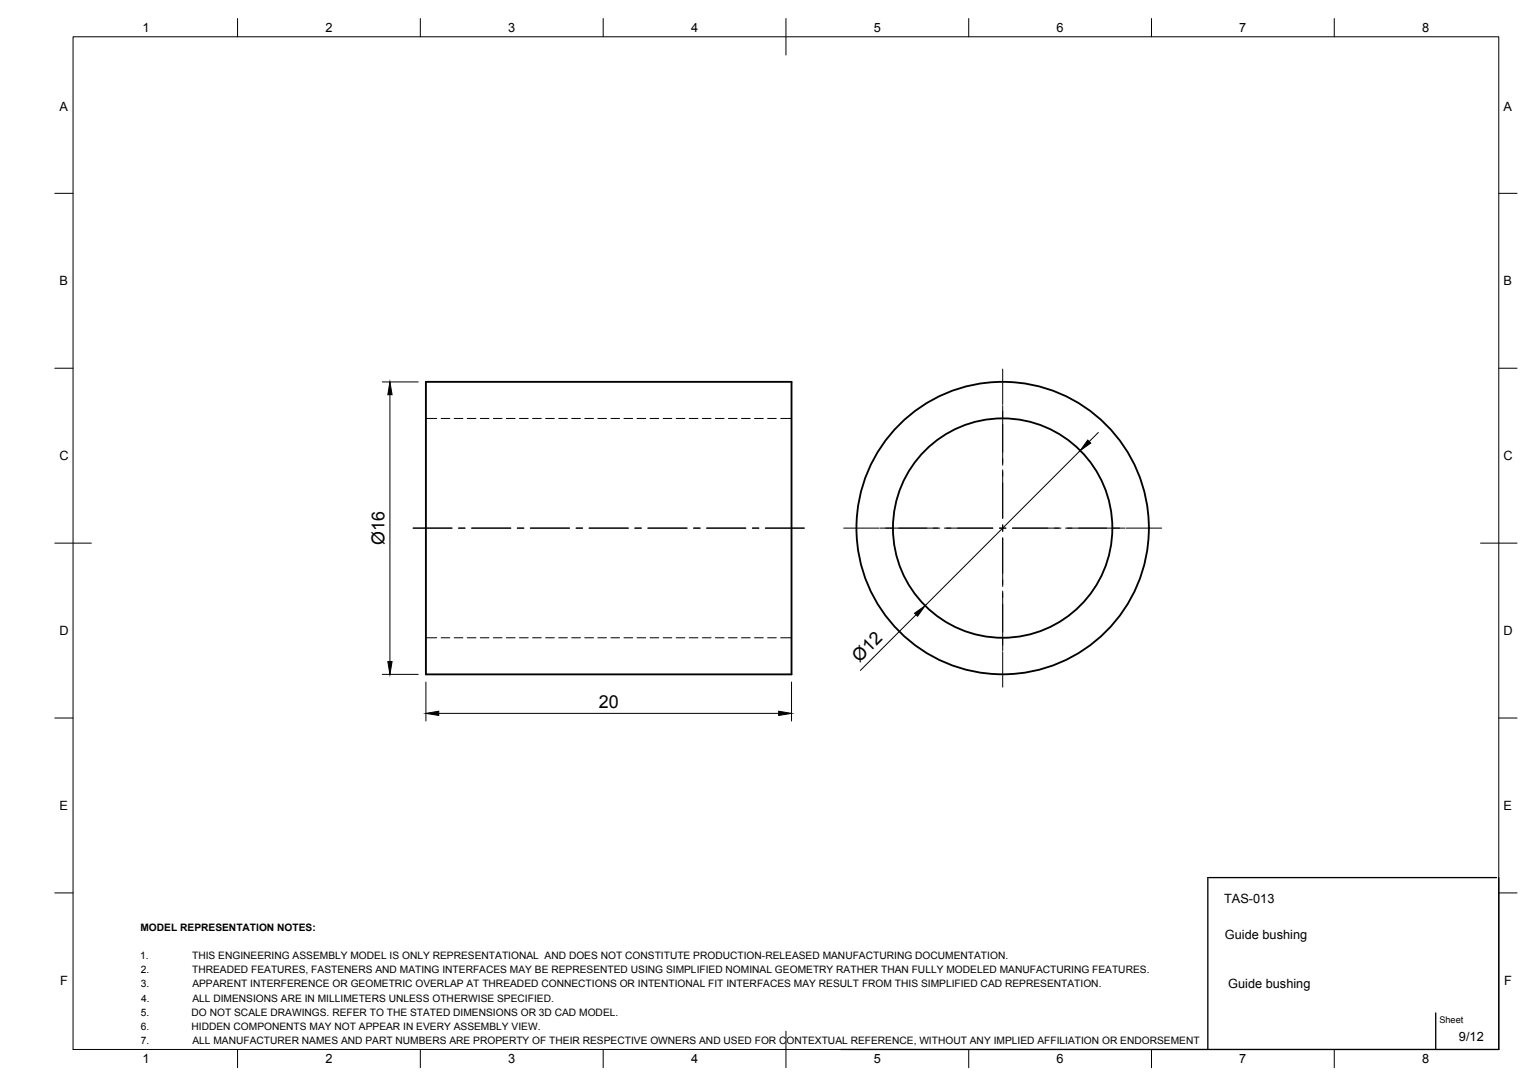
ISO-10303-21;
HEADER;
/* Generated by software containing ST-Developer
 * from STEP Tools, Inc. (www.steptools.com) 
 */

FILE_DESCRIPTION(
/* description */ (
'Independent guided parallel-jaw bracket clamp. Two12mm guide rods, re
placeable bronze sleeves, captured swiveling spindle, replaceable jaw 
pads and modeled M16x2 screw. Native slider/revolute joints linked2mm 
per revolution. Nominal opening0..122 with initial28mm. Base and two i
dentical supports welded. Standard fits, weld details and clamp load r
equire engineering selection.'),
/* implementation_level */ '2;1');

FILE_NAME(
/* name */ 'Guide bushing.step',
/* time_stamp */ '2026-11-14T09:15:44-08:00',
/* author */ (''),
/* organization */ (''),
/* preprocessor_version */ 'ST-DEVELOPER v20.2',
/* originating_system */ 'Autodesk Translation Framework v15.17.0.0',
/* authorisation */ '');

FILE_SCHEMA (('AUTOMOTIVE_DESIGN { 1 0 10303 214 3 1 1 }'));
ENDSEC;

DATA;
#10=MECHANICAL_DESIGN_GEOMETRIC_PRESENTATION_REPRESENTATION('',(#924),#105806);
#900=SHAPE_REPRESENTATION_RELATIONSHIP('SRR','None',#105868,#912);
#912=ADVANCED_BREP_SHAPE_REPRESENTATION('',(#936),#105803);
#924=STYLED_ITEM('',(#105930),#936);
#936=MANIFOLD_SOLID_BREP('Body1',#7211);
#992=FACE_BOUND('',#1617,.T.);
#993=FACE_BOUND('',#1619,.T.);
#1051=PLANE('',#7665);
#1052=PLANE('',#7666);
#1289=FACE_OUTER_BOUND('',#1614,.T.);
#1290=FACE_OUTER_BOUND('',#1615,.T.);
#1291=FACE_OUTER_BOUND('',#1616,.T.);
#1292=FACE_OUTER_BOUND('',#1618,.T.);
#1614=EDGE_LOOP('',(#6341,#6342,#6343,#6344));
#1615=EDGE_LOOP('',(#6345,#6346,#6347,#6348));
#1616=EDGE_LOOP('',(#6349));
#1617=EDGE_LOOP('',(#6350));
#1618=EDGE_LOOP('',(#6351));
#1619=EDGE_LOOP('',(#6352));
#1900=LINE('',#88827,#2180);
#1901=LINE('',#88833,#2181);
#2180=VECTOR('',#8603,6.);
#2181=VECTOR('',#8610,8.);
#2311=CIRCLE('',#7660,6.);
#2312=CIRCLE('',#7661,6.);
#2313=CIRCLE('',#7663,8.);
#2314=CIRCLE('',#7664,8.);
#3093=VERTEX_POINT('',#88824);
#3094=VERTEX_POINT('',#88826);
#3095=VERTEX_POINT('',#88830);
#3096=VERTEX_POINT('',#88832);
#4215=EDGE_CURVE('',#3093,#3093,#2311,.T.);
#4216=EDGE_CURVE('',#3093,#3094,#1900,.T.);
#4217=EDGE_CURVE('',#3094,#3094,#2312,.T.);
#4218=EDGE_CURVE('',#3095,#3095,#2313,.T.);
#4219=EDGE_CURVE('',#3095,#3096,#1901,.T.);
#4220=EDGE_CURVE('',#3096,#3096,#2314,.T.);
#6341=ORIENTED_EDGE('',*,*,#4215,.T.);
#6342=ORIENTED_EDGE('',*,*,#4216,.T.);
#6343=ORIENTED_EDGE('',*,*,#4217,.F.);
#6344=ORIENTED_EDGE('',*,*,#4216,.F.);
#6345=ORIENTED_EDGE('',*,*,#4218,.F.);
#6346=ORIENTED_EDGE('',*,*,#4219,.T.);
#6347=ORIENTED_EDGE('',*,*,#4220,.T.);
#6348=ORIENTED_EDGE('',*,*,#4219,.F.);
#6349=ORIENTED_EDGE('',*,*,#4218,.T.);
#6350=ORIENTED_EDGE('',*,*,#4217,.T.);
#6351=ORIENTED_EDGE('',*,*,#4220,.F.);
#6352=ORIENTED_EDGE('',*,*,#4215,.F.);
#6899=CYLINDRICAL_SURFACE('',#7659,6.);
#6900=CYLINDRICAL_SURFACE('',#7662,8.);
#7154=ADVANCED_FACE('',(#1289),#6899,.F.);
#7155=ADVANCED_FACE('',(#1290),#6900,.T.);
#7156=ADVANCED_FACE('',(#1291,#992),#1051,.T.);
#7157=ADVANCED_FACE('',(#1292,#993),#1052,.F.);
#7211=CLOSED_SHELL('',(#7154,#7155,#7156,#7157));
#7658=AXIS2_PLACEMENT_3D('',#88822,#8597,#8598);
#7659=AXIS2_PLACEMENT_3D('',#88823,#8599,#8600);
#7660=AXIS2_PLACEMENT_3D('',#88825,#8601,#8602);
#7661=AXIS2_PLACEMENT_3D('',#88828,#8604,#8605);
#7662=AXIS2_PLACEMENT_3D('',#88829,#8606,#8607);
#7663=AXIS2_PLACEMENT_3D('',#88831,#8608,#8609);
#7664=AXIS2_PLACEMENT_3D('',#88834,#8611,#8612);
#7665=AXIS2_PLACEMENT_3D('',#88835,#8613,#8614);
#7666=AXIS2_PLACEMENT_3D('',#88836,#8615,#8616);
#8597=DIRECTION('axis',(0.,0.,1.));
#8598=DIRECTION('refdir',(1.,0.,0.));
#8599=DIRECTION('center_axis',(0.,0.,1.));
#8600=DIRECTION('ref_axis',(1.,0.,0.));
#8601=DIRECTION('center_axis',(0.,0.,-1.));
#8602=DIRECTION('ref_axis',(1.,0.,0.));
#8603=DIRECTION('',(0.,0.,1.));
#8604=DIRECTION('center_axis',(0.,0.,-1.));
#8605=DIRECTION('ref_axis',(1.,0.,0.));
#8606=DIRECTION('center_axis',(0.,0.,1.));
#8607=DIRECTION('ref_axis',(1.,0.,0.));
#8608=DIRECTION('center_axis',(0.,0.,1.));
#8609=DIRECTION('ref_axis',(1.,0.,0.));
#8610=DIRECTION('',(0.,0.,-1.));
#8611=DIRECTION('center_axis',(0.,0.,1.));
#8612=DIRECTION('ref_axis',(1.,0.,0.));
#8613=DIRECTION('center_axis',(0.,0.,1.));
#8614=DIRECTION('ref_axis',(1.,0.,0.));
#8615=DIRECTION('center_axis',(0.,0.,1.));
#8616=DIRECTION('ref_axis',(1.,0.,0.));
#88822=CARTESIAN_POINT('',(0.,0.,0.));
#88823=CARTESIAN_POINT('Origin',(0.,0.,0.));
#88824=CARTESIAN_POINT('',(-6.,-7.34788079488412E-16,0.));
#88825=CARTESIAN_POINT('Origin',(0.,0.,0.));
#88826=CARTESIAN_POINT('',(-6.,-7.34788079488412E-16,20.));
#88827=CARTESIAN_POINT('',(-6.,-7.34788079488412E-16,0.));
#88828=CARTESIAN_POINT('Origin',(0.,0.,20.));
#88829=CARTESIAN_POINT('Origin',(0.,0.,0.));
#88830=CARTESIAN_POINT('',(-8.,-9.79717439317883E-16,20.));
#88831=CARTESIAN_POINT('Origin',(0.,0.,20.));
#88832=CARTESIAN_POINT('',(-8.,-9.79717439317883E-16,0.));
#88833=CARTESIAN_POINT('',(-8.,-9.79717439317883E-16,0.));
#88834=CARTESIAN_POINT('Origin',(0.,0.,0.));
#88835=CARTESIAN_POINT('Origin',(0.,0.,20.));
#88836=CARTESIAN_POINT('Origin',(0.,0.,0.));
#105789=UNCERTAINTY_MEASURE_WITH_UNIT(LENGTH_MEASURE(0.01),#105807,
'DISTANCE_ACCURACY_VALUE',
'Maximum model space distance between geometric entities at asserted c
onnectivities');
#105792=UNCERTAINTY_MEASURE_WITH_UNIT(LENGTH_MEASURE(0.01),#105807,
'DISTANCE_ACCURACY_VALUE',
'Maximum model space distance between geometric entities at asserted c
onnectivities');
#105803=(
GEOMETRIC_REPRESENTATION_CONTEXT(3)
GLOBAL_UNCERTAINTY_ASSIGNED_CONTEXT((#105789))
GLOBAL_UNIT_ASSIGNED_CONTEXT((#105807,#105809,#105810))
REPRESENTATION_CONTEXT('','3D')
);
#105806=(
GEOMETRIC_REPRESENTATION_CONTEXT(3)
GLOBAL_UNCERTAINTY_ASSIGNED_CONTEXT((#105792))
GLOBAL_UNIT_ASSIGNED_CONTEXT((#105807,#105809,#105810))
REPRESENTATION_CONTEXT('','3D')
);
#105807=(
LENGTH_UNIT()
NAMED_UNIT(*)
SI_UNIT(.MILLI.,.METRE.)
);
#105809=(
NAMED_UNIT(*)
PLANE_ANGLE_UNIT()
SI_UNIT($,.RADIAN.)
);
#105810=(
NAMED_UNIT(*)
SI_UNIT($,.STERADIAN.)
SOLID_ANGLE_UNIT()
);
#105821=SHAPE_DEFINITION_REPRESENTATION(#105834,#105868);
#105834=PRODUCT_DEFINITION_SHAPE('',$,#105882);
#105868=SHAPE_REPRESENTATION('',(#7658),#105803);
#105871=PRODUCT_DEFINITION_CONTEXT('part definition',#105912,'design');
#105882=PRODUCT_DEFINITION('Guide bushing','Guide bushing',#105895,#105871);
#105895=PRODUCT_DEFINITION_FORMATION('',$,#105924);
#105912=APPLICATION_CONTEXT(
'Core Data for Automotive Mechanical Design Process');
#105913=PRODUCT_CONTEXT('part definition',#105912,'mechanical');
#105924=PRODUCT('Guide bushing','Guide bushing',$,(#105913));
#105930=PRESENTATION_STYLE_ASSIGNMENT((#105936));
#105936=SURFACE_STYLE_USAGE(.BOTH.,#105942);
#105942=SURFACE_SIDE_STYLE('',(#105948));
#105948=SURFACE_STYLE_FILL_AREA(#105954);
#105954=FILL_AREA_STYLE('Opaque(185,192,202)',(#105960));
#105960=FILL_AREA_STYLE_COLOUR('Opaque(185,192,202)',#105966);
#105966=COLOUR_RGB('Opaque(185,192,202)',0.725490196078431,0.752941176470588,
0.792156862745098);
ENDSEC;
END-ISO-10303-21;
